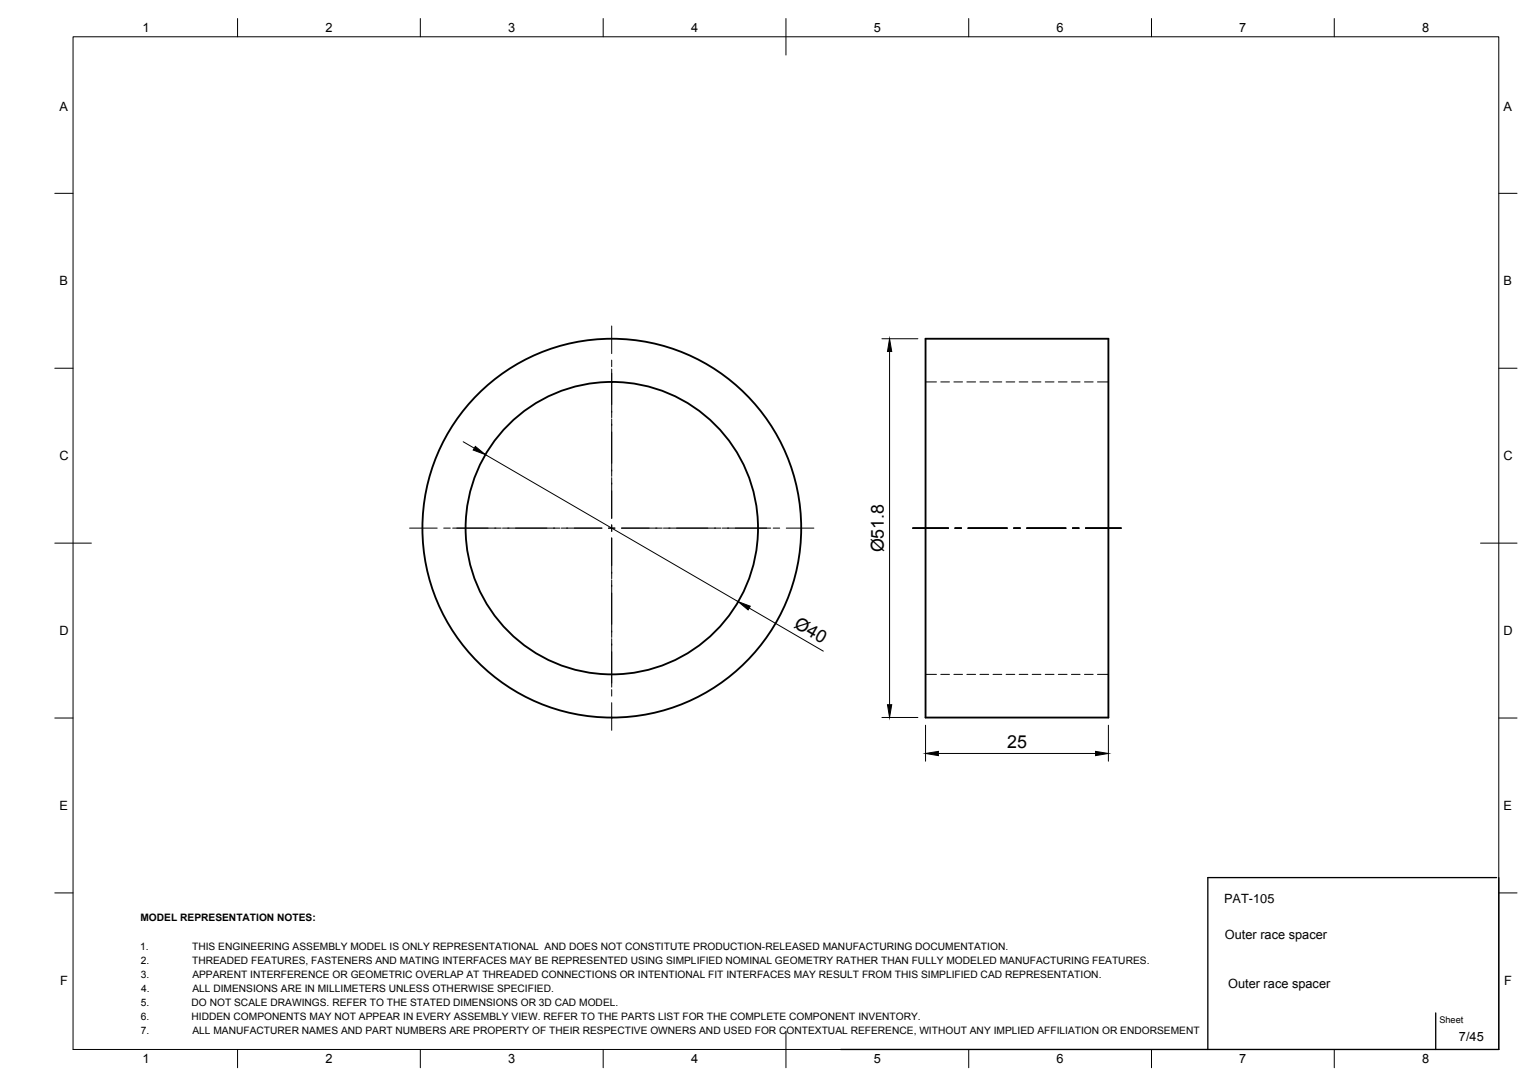
ISO-10303-21;
HEADER;
/* Generated by software containing ST-Developer
 * from STEP Tools, Inc. (www.steptools.com) 
 */

FILE_DESCRIPTION(
/* description */ ('Torque wrench calibration arm'),
/* implementation_level */ '2;1');

FILE_NAME(
/* name */ 'Outer race spacer.step',
/* time_stamp */ '2026-10-28T03:24:52-07:00',
/* author */ (''),
/* organization */ (''),
/* preprocessor_version */ 'ST-DEVELOPER v20.2',
/* originating_system */ 'Autodesk Translation Framework v15.17.0.0',
/* authorisation */ '');

FILE_SCHEMA (('AUTOMOTIVE_DESIGN { 1 0 10303 214 3 1 1 }'));
ENDSEC;

DATA;
#10=MECHANICAL_DESIGN_GEOMETRIC_PRESENTATION_REPRESENTATION('',(#428),#12783);
#354=SHAPE_REPRESENTATION_RELATIONSHIP('SRR','None',#12935,#391);
#391=ADVANCED_BREP_SHAPE_REPRESENTATION('',(#482),#12744);
#428=STYLED_ITEM('',(#13212),#482);
#482=MANIFOLD_SOLID_BREP('Body1',#6497);
#559=FACE_BOUND('',#1365,.T.);
#560=FACE_BOUND('',#1367,.T.);
#690=PLANE('',#7091);
#691=PLANE('',#7092);
#939=FACE_OUTER_BOUND('',#1362,.T.);
#940=FACE_OUTER_BOUND('',#1363,.T.);
#941=FACE_OUTER_BOUND('',#1364,.T.);
#942=FACE_OUTER_BOUND('',#1366,.T.);
#1362=EDGE_LOOP('',(#4651,#4652,#4653,#4654));
#1363=EDGE_LOOP('',(#4655,#4656,#4657,#4658));
#1364=EDGE_LOOP('',(#4659));
#1365=EDGE_LOOP('',(#4660));
#1366=EDGE_LOOP('',(#4661));
#1367=EDGE_LOOP('',(#4662));
#1880=LINE('',#10248,#2295);
#1881=LINE('',#10254,#2296);
#2295=VECTOR('',#8158,2.);
#2296=VECTOR('',#8165,2.59);
#2672=CIRCLE('',#7086,2.);
#2673=CIRCLE('',#7087,2.);
#2674=CIRCLE('',#7089,2.59);
#2675=CIRCLE('',#7090,2.59);
#3071=VERTEX_POINT('',#10245);
#3072=VERTEX_POINT('',#10247);
#3073=VERTEX_POINT('',#10251);
#3074=VERTEX_POINT('',#10253);
#3683=EDGE_CURVE('',#3071,#3071,#2672,.T.);
#3684=EDGE_CURVE('',#3071,#3072,#1880,.T.);
#3685=EDGE_CURVE('',#3072,#3072,#2673,.T.);
#3686=EDGE_CURVE('',#3073,#3073,#2674,.T.);
#3687=EDGE_CURVE('',#3073,#3074,#1881,.T.);
#3688=EDGE_CURVE('',#3074,#3074,#2675,.T.);
#4651=ORIENTED_EDGE('',*,*,#3683,.F.);
#4652=ORIENTED_EDGE('',*,*,#3684,.T.);
#4653=ORIENTED_EDGE('',*,*,#3685,.T.);
#4654=ORIENTED_EDGE('',*,*,#3684,.F.);
#4655=ORIENTED_EDGE('',*,*,#3686,.F.);
#4656=ORIENTED_EDGE('',*,*,#3687,.T.);
#4657=ORIENTED_EDGE('',*,*,#3688,.T.);
#4658=ORIENTED_EDGE('',*,*,#3687,.F.);
#4659=ORIENTED_EDGE('',*,*,#3686,.T.);
#4660=ORIENTED_EDGE('',*,*,#3683,.T.);
#4661=ORIENTED_EDGE('',*,*,#3688,.F.);
#4662=ORIENTED_EDGE('',*,*,#3685,.F.);
#6013=CYLINDRICAL_SURFACE('',#7085,2.);
#6014=CYLINDRICAL_SURFACE('',#7088,2.59);
#6164=ADVANCED_FACE('',(#939),#6013,.F.);
#6165=ADVANCED_FACE('',(#940),#6014,.T.);
#6166=ADVANCED_FACE('',(#941,#559),#690,.T.);
#6167=ADVANCED_FACE('',(#942,#560),#691,.F.);
#6497=CLOSED_SHELL('',(#6164,#6165,#6166,#6167));
#7084=AXIS2_PLACEMENT_3D('',#10243,#8152,#8153);
#7085=AXIS2_PLACEMENT_3D('',#10244,#8154,#8155);
#7086=AXIS2_PLACEMENT_3D('',#10246,#8156,#8157);
#7087=AXIS2_PLACEMENT_3D('',#10249,#8159,#8160);
#7088=AXIS2_PLACEMENT_3D('',#10250,#8161,#8162);
#7089=AXIS2_PLACEMENT_3D('',#10252,#8163,#8164);
#7090=AXIS2_PLACEMENT_3D('',#10255,#8166,#8167);
#7091=AXIS2_PLACEMENT_3D('',#10256,#8168,#8169);
#7092=AXIS2_PLACEMENT_3D('',#10257,#8170,#8171);
#8152=DIRECTION('axis',(0.,0.,1.));
#8153=DIRECTION('refdir',(1.,0.,0.));
#8154=DIRECTION('center_axis',(0.,1.,0.));
#8155=DIRECTION('ref_axis',(1.,0.,0.));
#8156=DIRECTION('center_axis',(0.,-1.,0.));
#8157=DIRECTION('ref_axis',(1.,0.,0.));
#8158=DIRECTION('',(0.,-1.,0.));
#8159=DIRECTION('center_axis',(0.,-1.,0.));
#8160=DIRECTION('ref_axis',(1.,0.,0.));
#8161=DIRECTION('center_axis',(0.,1.,0.));
#8162=DIRECTION('ref_axis',(1.,0.,0.));
#8163=DIRECTION('center_axis',(0.,1.,0.));
#8164=DIRECTION('ref_axis',(1.,0.,0.));
#8165=DIRECTION('',(0.,-1.,0.));
#8166=DIRECTION('center_axis',(0.,1.,0.));
#8167=DIRECTION('ref_axis',(1.,0.,0.));
#8168=DIRECTION('center_axis',(0.,1.,0.));
#8169=DIRECTION('ref_axis',(1.,0.,0.));
#8170=DIRECTION('center_axis',(0.,1.,0.));
#8171=DIRECTION('ref_axis',(1.,0.,0.));
#10243=CARTESIAN_POINT('',(0.,0.,0.));
#10244=CARTESIAN_POINT('Origin',(0.,1.75,8.));
#10245=CARTESIAN_POINT('',(-2.,4.25,8.));
#10246=CARTESIAN_POINT('Origin',(0.,4.25,8.));
#10247=CARTESIAN_POINT('',(-2.,1.75,8.));
#10248=CARTESIAN_POINT('',(-2.,1.75,8.));
#10249=CARTESIAN_POINT('Origin',(0.,1.75,8.));
#10250=CARTESIAN_POINT('Origin',(0.,1.75,8.));
#10251=CARTESIAN_POINT('',(-2.59,4.25,8.));
#10252=CARTESIAN_POINT('Origin',(0.,4.25,8.));
#10253=CARTESIAN_POINT('',(-2.59,1.75,8.));
#10254=CARTESIAN_POINT('',(-2.59,1.75,8.));
#10255=CARTESIAN_POINT('Origin',(0.,1.75,8.));
#10256=CARTESIAN_POINT('Origin',(0.,4.25,8.));
#10257=CARTESIAN_POINT('Origin',(0.,1.75,8.));
#12700=UNCERTAINTY_MEASURE_WITH_UNIT(LENGTH_MEASURE(0.001),#12784,
'DISTANCE_ACCURACY_VALUE',
'Maximum model space distance between geometric entities at asserted c
onnectivities');
#12739=UNCERTAINTY_MEASURE_WITH_UNIT(LENGTH_MEASURE(0.001),#12784,
'DISTANCE_ACCURACY_VALUE',
'Maximum model space distance between geometric entities at asserted c
onnectivities');
#12744=(
GEOMETRIC_REPRESENTATION_CONTEXT(3)
GLOBAL_UNCERTAINTY_ASSIGNED_CONTEXT((#12700))
GLOBAL_UNIT_ASSIGNED_CONTEXT((#12784,#12786,#12787))
REPRESENTATION_CONTEXT('','3D')
);
#12783=(
GEOMETRIC_REPRESENTATION_CONTEXT(3)
GLOBAL_UNCERTAINTY_ASSIGNED_CONTEXT((#12739))
GLOBAL_UNIT_ASSIGNED_CONTEXT((#12784,#12786,#12787))
REPRESENTATION_CONTEXT('','3D')
);
#12784=(
LENGTH_UNIT()
NAMED_UNIT(*)
SI_UNIT(.CENTI.,.METRE.)
);
#12786=(
NAMED_UNIT(*)
PLANE_ANGLE_UNIT()
SI_UNIT($,.RADIAN.)
);
#12787=(
NAMED_UNIT(*)
SI_UNIT($,.STERADIAN.)
SOLID_ANGLE_UNIT()
);
#12792=SHAPE_DEFINITION_REPRESENTATION(#12835,#12935);
#12835=PRODUCT_DEFINITION_SHAPE('',$,#12979);
#12935=SHAPE_REPRESENTATION('',(#7084),#12744);
#12974=PRODUCT_DEFINITION_CONTEXT('part definition',#13105,'design');
#12979=PRODUCT_DEFINITION('Outer race spacer','Outer race spacer',#13022,
#12974);
#13022=PRODUCT_DEFINITION_FORMATION('',$,#13111);
#13105=APPLICATION_CONTEXT(
'Core Data for Automotive Mechanical Design Process');
#13106=PRODUCT_CONTEXT('part definition',#13105,'mechanical');
#13111=PRODUCT('Outer race spacer','Outer race spacer',
'Outer race spacer',(#13106));
#13206=COLOUR_RGB('Grey',0.48,0.52,0.57);
#13207=FILL_AREA_STYLE_COLOUR('',#13206);
#13208=FILL_AREA_STYLE('',(#13207));
#13209=SURFACE_STYLE_FILL_AREA(#13208);
#13210=SURFACE_SIDE_STYLE('',(#13209));
#13211=SURFACE_STYLE_USAGE(.BOTH.,#13210);
#13212=PRESENTATION_STYLE_ASSIGNMENT((#13211));
ENDSEC;
END-ISO-10303-21;
